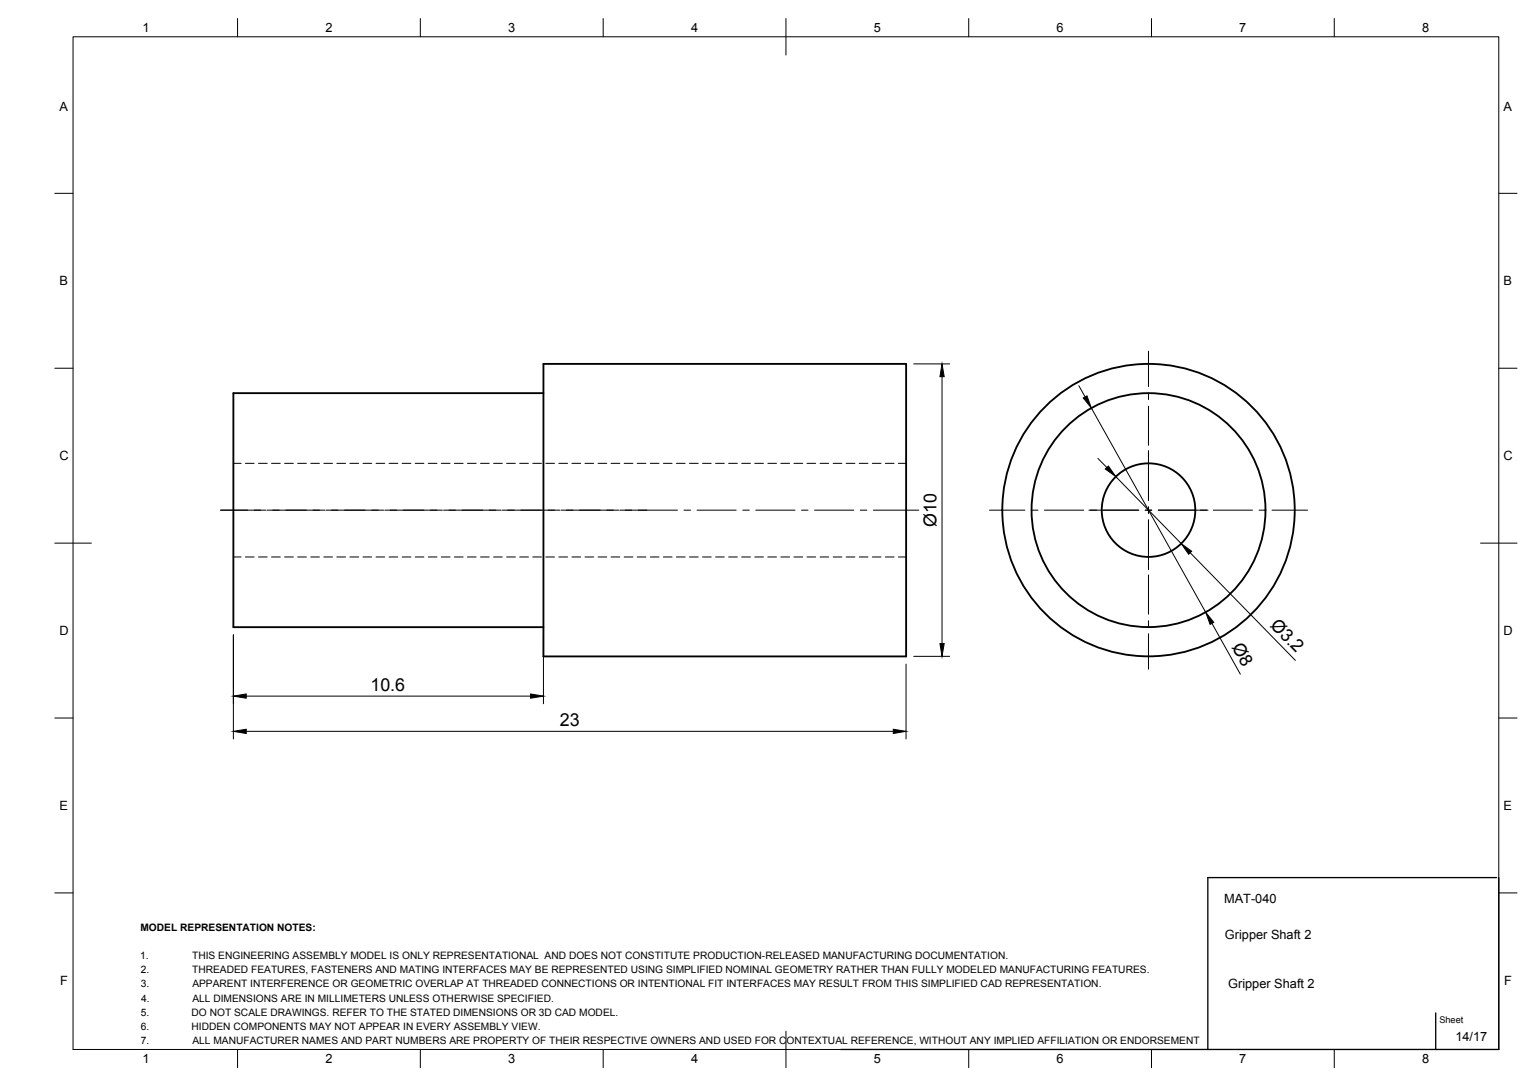
ISO-10303-21;
HEADER;
/* Generated by software containing ST-Developer
 * from STEP Tools, Inc. (www.steptools.com) 
 */

FILE_DESCRIPTION(
/* description */ ('STEP AP214'),
/* implementation_level */ '2;1');

FILE_NAME(
/* name */ 'Gripper Shaft 2.step',
/* time_stamp */ '2026-11-14T21:53:28-08:00',
/* author */ (''),
/* organization */ (''),
/* preprocessor_version */ 'ST-DEVELOPER v20.2',
/* originating_system */ 'Autodesk Translation Framework v15.17.0.0',
/* authorisation */ '');

FILE_SCHEMA (('AUTOMOTIVE_DESIGN { 1 0 10303 214 3 1 1 }'));
ENDSEC;

DATA;
#10=MECHANICAL_DESIGN_GEOMETRIC_PRESENTATION_REPRESENTATION('',(#350),#20176);
#303=SHAPE_REPRESENTATION_RELATIONSHIP('SRR','None',#20267,#315);
#315=ADVANCED_BREP_SHAPE_REPRESENTATION('',(#377),#20173);
#350=STYLED_ITEM('',(#20337),#377);
#377=MANIFOLD_SOLID_BREP('Body1',#10968);
#568=FACE_BOUND('',#2240,.T.);
#569=FACE_BOUND('',#2242,.T.);
#570=FACE_BOUND('',#2244,.T.);
#879=PLANE('',#12112);
#880=PLANE('',#12113);
#881=PLANE('',#12114);
#1456=FACE_OUTER_BOUND('',#2236,.T.);
#1457=FACE_OUTER_BOUND('',#2237,.T.);
#1458=FACE_OUTER_BOUND('',#2238,.T.);
#1459=FACE_OUTER_BOUND('',#2239,.T.);
#1460=FACE_OUTER_BOUND('',#2241,.T.);
#1461=FACE_OUTER_BOUND('',#2243,.T.);
#2236=EDGE_LOOP('',(#9999,#10000,#10001,#10002));
#2237=EDGE_LOOP('',(#10003,#10004,#10005,#10006));
#2238=EDGE_LOOP('',(#10007,#10008,#10009,#10010));
#2239=EDGE_LOOP('',(#10011));
#2240=EDGE_LOOP('',(#10012));
#2241=EDGE_LOOP('',(#10013));
#2242=EDGE_LOOP('',(#10014));
#2243=EDGE_LOOP('',(#10015));
#2244=EDGE_LOOP('',(#10016));
#3224=LINE('',#19949,#4212);
#3225=LINE('',#19955,#4213);
#3226=LINE('',#19961,#4214);
#4212=VECTOR('',#15160,5.);
#4213=VECTOR('',#15167,1.6);
#4214=VECTOR('',#15174,4.);
#4698=CIRCLE('',#12104,5.);
#4699=CIRCLE('',#12105,5.);
#4700=CIRCLE('',#12107,1.6);
#4701=CIRCLE('',#12108,1.6);
#4702=CIRCLE('',#12110,4.);
#4703=CIRCLE('',#12111,4.);
#5649=VERTEX_POINT('',#19946);
#5650=VERTEX_POINT('',#19948);
#5651=VERTEX_POINT('',#19952);
#5652=VERTEX_POINT('',#19954);
#5653=VERTEX_POINT('',#19958);
#5654=VERTEX_POINT('',#19960);
#7110=EDGE_CURVE('',#5649,#5649,#4698,.T.);
#7111=EDGE_CURVE('',#5649,#5650,#3224,.T.);
#7112=EDGE_CURVE('',#5650,#5650,#4699,.T.);
#7113=EDGE_CURVE('',#5651,#5651,#4700,.T.);
#7114=EDGE_CURVE('',#5651,#5652,#3225,.T.);
#7115=EDGE_CURVE('',#5652,#5652,#4701,.T.);
#7116=EDGE_CURVE('',#5653,#5653,#4702,.T.);
#7117=EDGE_CURVE('',#5653,#5654,#3226,.T.);
#7118=EDGE_CURVE('',#5654,#5654,#4703,.T.);
#9999=ORIENTED_EDGE('',*,*,#7110,.F.);
#10000=ORIENTED_EDGE('',*,*,#7111,.T.);
#10001=ORIENTED_EDGE('',*,*,#7112,.T.);
#10002=ORIENTED_EDGE('',*,*,#7111,.F.);
#10003=ORIENTED_EDGE('',*,*,#7113,.T.);
#10004=ORIENTED_EDGE('',*,*,#7114,.T.);
#10005=ORIENTED_EDGE('',*,*,#7115,.F.);
#10006=ORIENTED_EDGE('',*,*,#7114,.F.);
#10007=ORIENTED_EDGE('',*,*,#7116,.F.);
#10008=ORIENTED_EDGE('',*,*,#7117,.T.);
#10009=ORIENTED_EDGE('',*,*,#7118,.F.);
#10010=ORIENTED_EDGE('',*,*,#7117,.F.);
#10011=ORIENTED_EDGE('',*,*,#7118,.T.);
#10012=ORIENTED_EDGE('',*,*,#7113,.F.);
#10013=ORIENTED_EDGE('',*,*,#7110,.T.);
#10014=ORIENTED_EDGE('',*,*,#7115,.T.);
#10015=ORIENTED_EDGE('',*,*,#7112,.F.);
#10016=ORIENTED_EDGE('',*,*,#7116,.T.);
#10343=CYLINDRICAL_SURFACE('',#12103,5.);
#10344=CYLINDRICAL_SURFACE('',#12106,1.6);
#10345=CYLINDRICAL_SURFACE('',#12109,4.);
#10908=ADVANCED_FACE('',(#1456),#10343,.T.);
#10909=ADVANCED_FACE('',(#1457),#10344,.F.);
#10910=ADVANCED_FACE('',(#1458),#10345,.T.);
#10911=ADVANCED_FACE('',(#1459,#568),#879,.T.);
#10912=ADVANCED_FACE('',(#1460,#569),#880,.F.);
#10913=ADVANCED_FACE('',(#1461,#570),#881,.F.);
#10968=CLOSED_SHELL('',(#10908,#10909,#10910,#10911,#10912,#10913));
#12102=AXIS2_PLACEMENT_3D('',#19944,#15154,#15155);
#12103=AXIS2_PLACEMENT_3D('',#19945,#15156,#15157);
#12104=AXIS2_PLACEMENT_3D('',#19947,#15158,#15159);
#12105=AXIS2_PLACEMENT_3D('',#19950,#15161,#15162);
#12106=AXIS2_PLACEMENT_3D('',#19951,#15163,#15164);
#12107=AXIS2_PLACEMENT_3D('',#19953,#15165,#15166);
#12108=AXIS2_PLACEMENT_3D('',#19956,#15168,#15169);
#12109=AXIS2_PLACEMENT_3D('',#19957,#15170,#15171);
#12110=AXIS2_PLACEMENT_3D('',#19959,#15172,#15173);
#12111=AXIS2_PLACEMENT_3D('',#19962,#15175,#15176);
#12112=AXIS2_PLACEMENT_3D('',#19963,#15177,#15178);
#12113=AXIS2_PLACEMENT_3D('',#19964,#15179,#15180);
#12114=AXIS2_PLACEMENT_3D('',#19965,#15181,#15182);
#15154=DIRECTION('axis',(0.,0.,1.));
#15155=DIRECTION('refdir',(1.,0.,0.));
#15156=DIRECTION('center_axis',(6.16297582203916E-33,-5.54667823983524E-32,
-1.));
#15157=DIRECTION('ref_axis',(-1.,-6.66133814775094E-16,-6.16297582203912E-33));
#15158=DIRECTION('center_axis',(6.16297582203915E-33,-6.77927340424307E-32,
-1.));
#15159=DIRECTION('ref_axis',(-1.,-6.66133814775094E-16,-6.16297582203911E-33));
#15160=DIRECTION('',(-6.16297582203916E-33,5.54667823983524E-32,1.));
#15161=DIRECTION('center_axis',(6.16297582203915E-33,-6.77927340424307E-32,
-1.));
#15162=DIRECTION('ref_axis',(-1.,-6.66133814775094E-16,-6.16297582203911E-33));
#15163=DIRECTION('center_axis',(6.16297582203915E-33,-6.77927340424307E-32,
-1.));
#15164=DIRECTION('ref_axis',(-1.,-6.66133814775094E-16,-6.16297582203911E-33));
#15165=DIRECTION('center_axis',(-6.16297582203915E-33,6.77927340424307E-32,
1.));
#15166=DIRECTION('ref_axis',(1.,6.66133814775094E-16,6.16297582203911E-33));
#15167=DIRECTION('',(6.16297582203915E-33,-6.77927340424307E-32,-1.));
#15168=DIRECTION('center_axis',(-6.16297582203915E-33,6.77927340424307E-32,
1.));
#15169=DIRECTION('ref_axis',(1.,6.66133814775094E-16,6.16297582203911E-33));
#15170=DIRECTION('center_axis',(6.16297582203915E-33,-6.77927340424307E-32,
-1.));
#15171=DIRECTION('ref_axis',(-1.,-6.66133814775094E-16,-6.16297582203911E-33));
#15172=DIRECTION('center_axis',(6.16297582203915E-33,-6.77927340424307E-32,
-1.));
#15173=DIRECTION('ref_axis',(-1.,-6.66133814775094E-16,-6.16297582203911E-33));
#15174=DIRECTION('',(-6.16297582203915E-33,6.77927340424307E-32,1.));
#15175=DIRECTION('center_axis',(-6.16297582203915E-33,6.77927340424307E-32,
1.));
#15176=DIRECTION('ref_axis',(1.,6.66133814775094E-16,6.16297582203911E-33));
#15177=DIRECTION('center_axis',(1.54074395550978E-32,6.77927340424307E-32,
1.));
#15178=DIRECTION('ref_axis',(1.,6.66133814775094E-16,-1.54074395550979E-32));
#15179=DIRECTION('center_axis',(1.54074395550978E-32,6.77927340424307E-32,
1.));
#15180=DIRECTION('ref_axis',(1.,6.66133814775094E-16,-1.54074395550979E-32));
#15181=DIRECTION('center_axis',(-1.54074395550978E-32,-6.77927340424307E-32,
-1.));
#15182=DIRECTION('ref_axis',(-1.,-6.66133814775094E-16,1.54074395550979E-32));
#19944=CARTESIAN_POINT('',(0.,0.,0.));
#19945=CARTESIAN_POINT('Origin',(-4.33680868994202E-15,-2.08166817117217E-14,
12.4));
#19946=CARTESIAN_POINT('',(4.99999999999999,-1.80983360374199E-14,0.));
#19947=CARTESIAN_POINT('Origin',(0.,0.,0.));
#19948=CARTESIAN_POINT('',(4.99999999999999,-1.80983360374199E-14,12.4));
#19949=CARTESIAN_POINT('',(4.99999999999999,-1.80983360374199E-14,12.4));
#19950=CARTESIAN_POINT('Origin',(-4.33680868994202E-15,-2.08166817117217E-14,
12.4));
#19951=CARTESIAN_POINT('Origin',(-3.46944695195361E-15,-2.08166817117217E-14,
23.));
#19952=CARTESIAN_POINT('',(1.6,-1.99468110959451E-14,23.));
#19953=CARTESIAN_POINT('Origin',(-3.46944695195361E-15,-2.08166817117217E-14,
23.));
#19954=CARTESIAN_POINT('',(1.6,-1.99468110959451E-14,0.));
#19955=CARTESIAN_POINT('',(1.6,-1.99468110959451E-14,23.));
#19956=CARTESIAN_POINT('Origin',(0.,0.,0.));
#19957=CARTESIAN_POINT('Origin',(-3.46944695195361E-15,-2.08166817117217E-14,
23.));
#19958=CARTESIAN_POINT('',(4.,-1.86420051722803E-14,12.4));
#19959=CARTESIAN_POINT('Origin',(-4.33680868994202E-15,-2.08166817117217E-14,
12.4));
#19960=CARTESIAN_POINT('',(4.,-1.86420051722803E-14,23.));
#19961=CARTESIAN_POINT('',(4.,-1.86420051722803E-14,23.));
#19962=CARTESIAN_POINT('Origin',(-3.46944695195361E-15,-2.08166817117217E-14,
23.));
#19963=CARTESIAN_POINT('Origin',(-3.46944695195361E-15,-2.08166817117217E-14,
23.));
#19964=CARTESIAN_POINT('Origin',(0.,0.,0.));
#19965=CARTESIAN_POINT('Origin',(-4.33680868994202E-15,-2.08166817117217E-14,
12.4));
#20157=UNCERTAINTY_MEASURE_WITH_UNIT(LENGTH_MEASURE(0.01),#20177,
'DISTANCE_ACCURACY_VALUE',
'Maximum model space distance between geometric entities at asserted c
onnectivities');
#20160=UNCERTAINTY_MEASURE_WITH_UNIT(LENGTH_MEASURE(0.01),#20177,
'DISTANCE_ACCURACY_VALUE',
'Maximum model space distance between geometric entities at asserted c
onnectivities');
#20173=(
GEOMETRIC_REPRESENTATION_CONTEXT(3)
GLOBAL_UNCERTAINTY_ASSIGNED_CONTEXT((#20157))
GLOBAL_UNIT_ASSIGNED_CONTEXT((#20177,#20179,#20180))
REPRESENTATION_CONTEXT('','3D')
);
#20176=(
GEOMETRIC_REPRESENTATION_CONTEXT(3)
GLOBAL_UNCERTAINTY_ASSIGNED_CONTEXT((#20160))
GLOBAL_UNIT_ASSIGNED_CONTEXT((#20177,#20179,#20180))
REPRESENTATION_CONTEXT('','3D')
);
#20177=(
LENGTH_UNIT()
NAMED_UNIT(*)
SI_UNIT(.MILLI.,.METRE.)
);
#20179=(
NAMED_UNIT(*)
PLANE_ANGLE_UNIT()
SI_UNIT($,.RADIAN.)
);
#20180=(
NAMED_UNIT(*)
SI_UNIT($,.STERADIAN.)
SOLID_ANGLE_UNIT()
);
#20193=SHAPE_DEFINITION_REPRESENTATION(#20208,#20267);
#20208=PRODUCT_DEFINITION_SHAPE('',$,#20283);
#20267=SHAPE_REPRESENTATION('',(#12102),#20173);
#20270=PRODUCT_DEFINITION_CONTEXT('part definition',#20317,'design');
#20283=PRODUCT_DEFINITION('Gripper Shaft 2','Gripper Shaft 2',#20298,#20270);
#20298=PRODUCT_DEFINITION_FORMATION('',$,#20331);
#20317=APPLICATION_CONTEXT(
'Core Data for Automotive Mechanical Design Process');
#20318=PRODUCT_CONTEXT('part definition',#20317,'mechanical');
#20331=PRODUCT('Gripper Shaft 2','Gripper Shaft 2',$,(#20318));
#20337=PRESENTATION_STYLE_ASSIGNMENT((#20342));
#20342=SURFACE_STYLE_USAGE(.BOTH.,#20347);
#20347=SURFACE_SIDE_STYLE('',(#20352));
#20352=SURFACE_STYLE_FILL_AREA(#20357);
#20357=FILL_AREA_STYLE('Opaque(31,36,43)',(#20362));
#20362=FILL_AREA_STYLE_COLOUR('Opaque(31,36,43)',#20367);
#20367=COLOUR_RGB('Opaque(31,36,43)',0.12156862745098,0.141176470588235,
0.168627450980392);
ENDSEC;
END-ISO-10303-21;
